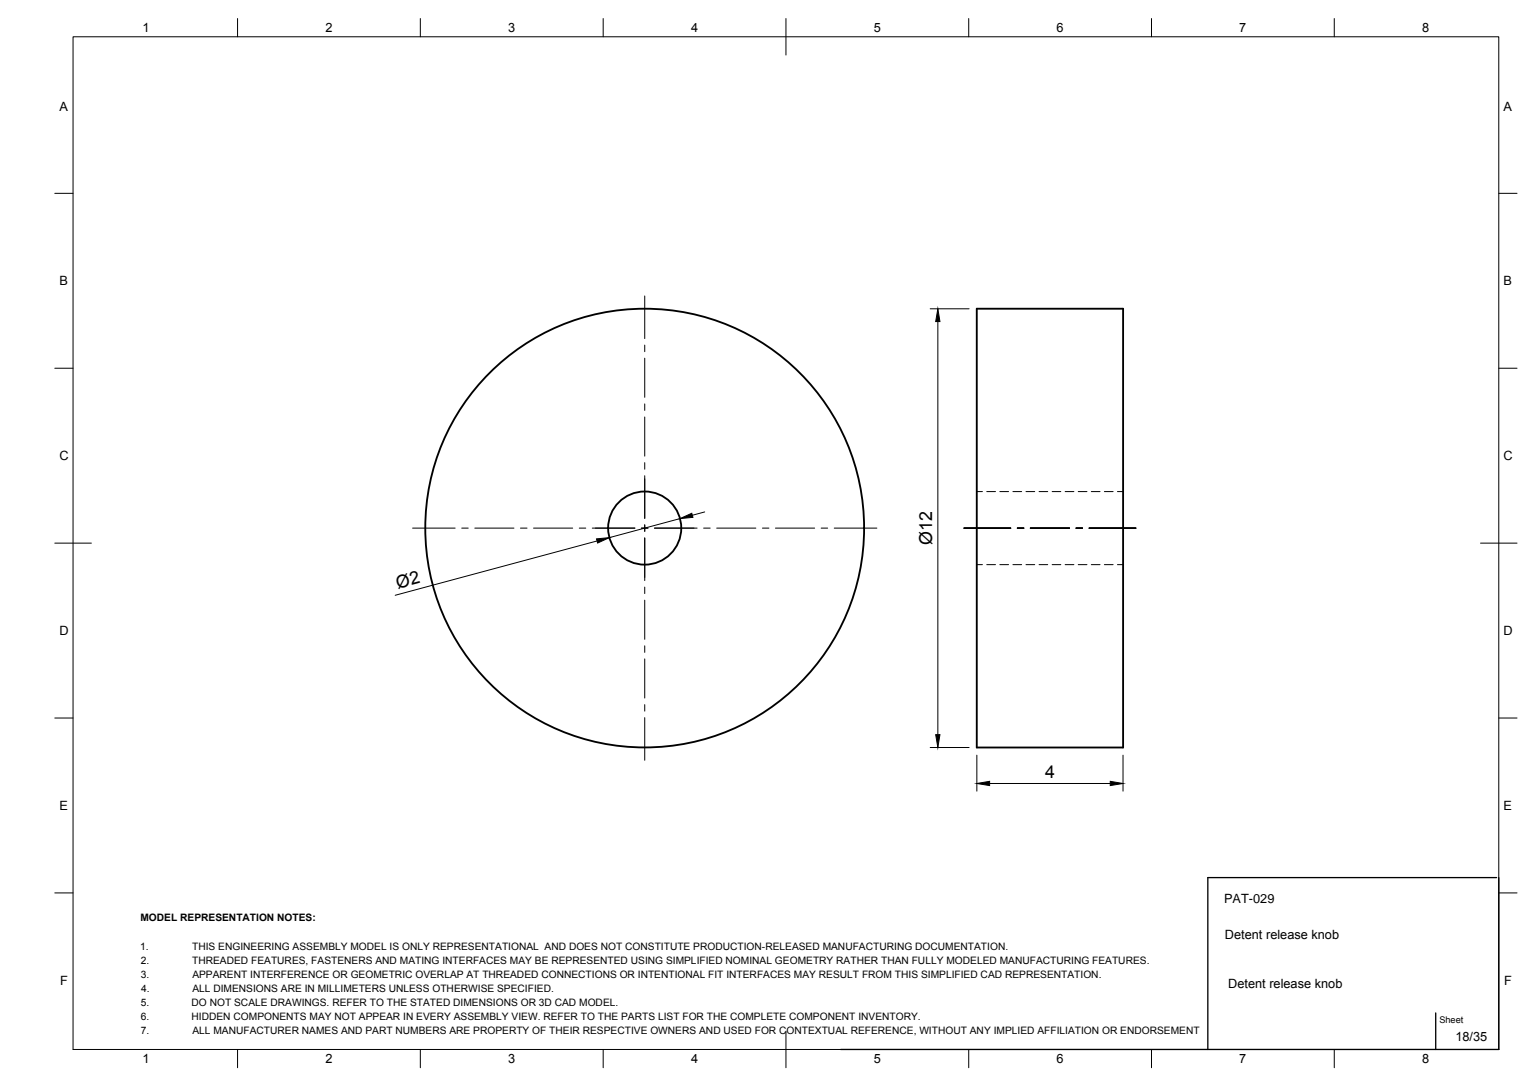
ISO-10303-21;
HEADER;
/* Generated by software containing ST-Developer
 * from STEP Tools, Inc. (www.steptools.com) 
 */

FILE_DESCRIPTION(
/* description */ ('Door-style hinge test fixture with detent'),
/* implementation_level */ '2;1');

FILE_NAME(
/* name */ 'Detent release knob.step',
/* time_stamp */ '2026-10-28T03:24:57-07:00',
/* author */ (''),
/* organization */ (''),
/* preprocessor_version */ 'ST-DEVELOPER v20.2',
/* originating_system */ 'Autodesk Translation Framework v15.17.0.0',
/* authorisation */ '');

FILE_SCHEMA (('AUTOMOTIVE_DESIGN { 1 0 10303 214 3 1 1 }'));
ENDSEC;

DATA;
#10=MECHANICAL_DESIGN_GEOMETRIC_PRESENTATION_REPRESENTATION('',(#336),#9813);
#273=SHAPE_REPRESENTATION_RELATIONSHIP('SRR','None',#9950,#304);
#304=ADVANCED_BREP_SHAPE_REPRESENTATION('',(#376),#9793);
#336=STYLED_ITEM('',(#10169),#376);
#376=MANIFOLD_SOLID_BREP('Body1',#4767);
#463=FACE_BOUND('',#1138,.T.);
#464=FACE_BOUND('',#1140,.T.);
#576=PLANE('',#5388);
#577=PLANE('',#5389);
#786=FACE_OUTER_BOUND('',#1135,.T.);
#787=FACE_OUTER_BOUND('',#1136,.T.);
#788=FACE_OUTER_BOUND('',#1137,.T.);
#789=FACE_OUTER_BOUND('',#1139,.T.);
#1135=EDGE_LOOP('',(#3761,#3762,#3763,#3764));
#1136=EDGE_LOOP('',(#3765,#3766,#3767,#3768));
#1137=EDGE_LOOP('',(#3769));
#1138=EDGE_LOOP('',(#3770));
#1139=EDGE_LOOP('',(#3771));
#1140=EDGE_LOOP('',(#3772));
#1506=LINE('',#7903,#1826);
#1507=LINE('',#7909,#1827);
#1826=VECTOR('',#6415,0.1);
#1827=VECTOR('',#6422,0.6);
#2079=CIRCLE('',#5383,0.1);
#2080=CIRCLE('',#5384,0.1);
#2081=CIRCLE('',#5386,0.6);
#2082=CIRCLE('',#5387,0.6);
#2407=VERTEX_POINT('',#7900);
#2408=VERTEX_POINT('',#7902);
#2409=VERTEX_POINT('',#7906);
#2410=VERTEX_POINT('',#7908);
#2897=EDGE_CURVE('',#2407,#2407,#2079,.T.);
#2898=EDGE_CURVE('',#2407,#2408,#1506,.T.);
#2899=EDGE_CURVE('',#2408,#2408,#2080,.T.);
#2900=EDGE_CURVE('',#2409,#2409,#2081,.T.);
#2901=EDGE_CURVE('',#2409,#2410,#1507,.T.);
#2902=EDGE_CURVE('',#2410,#2410,#2082,.T.);
#3761=ORIENTED_EDGE('',*,*,#2897,.F.);
#3762=ORIENTED_EDGE('',*,*,#2898,.T.);
#3763=ORIENTED_EDGE('',*,*,#2899,.T.);
#3764=ORIENTED_EDGE('',*,*,#2898,.F.);
#3765=ORIENTED_EDGE('',*,*,#2900,.F.);
#3766=ORIENTED_EDGE('',*,*,#2901,.T.);
#3767=ORIENTED_EDGE('',*,*,#2902,.T.);
#3768=ORIENTED_EDGE('',*,*,#2901,.F.);
#3769=ORIENTED_EDGE('',*,*,#2900,.T.);
#3770=ORIENTED_EDGE('',*,*,#2897,.T.);
#3771=ORIENTED_EDGE('',*,*,#2902,.F.);
#3772=ORIENTED_EDGE('',*,*,#2899,.F.);
#4427=CYLINDRICAL_SURFACE('',#5382,0.1);
#4428=CYLINDRICAL_SURFACE('',#5385,0.6);
#4591=ADVANCED_FACE('',(#786),#4427,.F.);
#4592=ADVANCED_FACE('',(#787),#4428,.T.);
#4593=ADVANCED_FACE('',(#788,#463),#576,.T.);
#4594=ADVANCED_FACE('',(#789,#464),#577,.F.);
#4767=CLOSED_SHELL('',(#4591,#4592,#4593,#4594));
#5381=AXIS2_PLACEMENT_3D('',#7898,#6409,#6410);
#5382=AXIS2_PLACEMENT_3D('',#7899,#6411,#6412);
#5383=AXIS2_PLACEMENT_3D('',#7901,#6413,#6414);
#5384=AXIS2_PLACEMENT_3D('',#7904,#6416,#6417);
#5385=AXIS2_PLACEMENT_3D('',#7905,#6418,#6419);
#5386=AXIS2_PLACEMENT_3D('',#7907,#6420,#6421);
#5387=AXIS2_PLACEMENT_3D('',#7910,#6423,#6424);
#5388=AXIS2_PLACEMENT_3D('',#7911,#6425,#6426);
#5389=AXIS2_PLACEMENT_3D('',#7912,#6427,#6428);
#6409=DIRECTION('axis',(0.,0.,1.));
#6410=DIRECTION('refdir',(1.,0.,0.));
#6411=DIRECTION('center_axis',(0.,1.,0.));
#6412=DIRECTION('ref_axis',(1.,0.,0.));
#6413=DIRECTION('center_axis',(0.,-1.,0.));
#6414=DIRECTION('ref_axis',(1.,0.,0.));
#6415=DIRECTION('',(0.,-1.,0.));
#6416=DIRECTION('center_axis',(0.,-1.,0.));
#6417=DIRECTION('ref_axis',(1.,0.,0.));
#6418=DIRECTION('center_axis',(0.,1.,0.));
#6419=DIRECTION('ref_axis',(1.,0.,0.));
#6420=DIRECTION('center_axis',(0.,1.,0.));
#6421=DIRECTION('ref_axis',(1.,0.,0.));
#6422=DIRECTION('',(0.,-1.,0.));
#6423=DIRECTION('center_axis',(0.,1.,0.));
#6424=DIRECTION('ref_axis',(1.,0.,0.));
#6425=DIRECTION('center_axis',(0.,1.,0.));
#6426=DIRECTION('ref_axis',(1.,0.,0.));
#6427=DIRECTION('center_axis',(0.,1.,0.));
#6428=DIRECTION('ref_axis',(1.,0.,0.));
#7898=CARTESIAN_POINT('',(0.,0.,0.));
#7899=CARTESIAN_POINT('Origin',(0.,-5.,7.2));
#7900=CARTESIAN_POINT('',(-0.1,-4.6,7.2));
#7901=CARTESIAN_POINT('Origin',(0.,-4.6,7.2));
#7902=CARTESIAN_POINT('',(-0.1,-5.,7.2));
#7903=CARTESIAN_POINT('',(-0.1,-5.,7.2));
#7904=CARTESIAN_POINT('Origin',(0.,-5.,7.2));
#7905=CARTESIAN_POINT('Origin',(0.,-5.,7.2));
#7906=CARTESIAN_POINT('',(-0.6,-4.6,7.2));
#7907=CARTESIAN_POINT('Origin',(0.,-4.6,7.2));
#7908=CARTESIAN_POINT('',(-0.6,-5.,7.2));
#7909=CARTESIAN_POINT('',(-0.6,-5.,7.2));
#7910=CARTESIAN_POINT('Origin',(0.,-5.,7.2));
#7911=CARTESIAN_POINT('Origin',(0.,-4.6,7.2));
#7912=CARTESIAN_POINT('Origin',(0.,-5.,7.2));
#9757=UNCERTAINTY_MEASURE_WITH_UNIT(LENGTH_MEASURE(0.001),#9814,
'DISTANCE_ACCURACY_VALUE',
'Maximum model space distance between geometric entities at asserted c
onnectivities');
#9777=UNCERTAINTY_MEASURE_WITH_UNIT(LENGTH_MEASURE(0.001),#9814,
'DISTANCE_ACCURACY_VALUE',
'Maximum model space distance between geometric entities at asserted c
onnectivities');
#9793=(
GEOMETRIC_REPRESENTATION_CONTEXT(3)
GLOBAL_UNCERTAINTY_ASSIGNED_CONTEXT((#9757))
GLOBAL_UNIT_ASSIGNED_CONTEXT((#9814,#9816,#9817))
REPRESENTATION_CONTEXT('','3D')
);
#9813=(
GEOMETRIC_REPRESENTATION_CONTEXT(3)
GLOBAL_UNCERTAINTY_ASSIGNED_CONTEXT((#9777))
GLOBAL_UNIT_ASSIGNED_CONTEXT((#9814,#9816,#9817))
REPRESENTATION_CONTEXT('','3D')
);
#9814=(
LENGTH_UNIT()
NAMED_UNIT(*)
SI_UNIT(.CENTI.,.METRE.)
);
#9816=(
NAMED_UNIT(*)
PLANE_ANGLE_UNIT()
SI_UNIT($,.RADIAN.)
);
#9817=(
NAMED_UNIT(*)
SI_UNIT($,.STERADIAN.)
SOLID_ANGLE_UNIT()
);
#9833=SHAPE_DEFINITION_REPRESENTATION(#9868,#9950);
#9868=PRODUCT_DEFINITION_SHAPE('',$,#9986);
#9950=SHAPE_REPRESENTATION('',(#5381),#9793);
#9970=PRODUCT_DEFINITION_CONTEXT('part definition',#10077,'design');
#9986=PRODUCT_DEFINITION('Detent release knob','Detent release knob',#10021,
#9970);
#10021=PRODUCT_DEFINITION_FORMATION('',$,#10094);
#10077=APPLICATION_CONTEXT(
'Core Data for Automotive Mechanical Design Process');
#10078=PRODUCT_CONTEXT('part definition',#10077,'mechanical');
#10094=PRODUCT('Detent release knob','Detent release knob',
'Detent release knob',(#10078));
#10163=COLOUR_RGB('Light Blue',0.38,0.62,0.78);
#10164=FILL_AREA_STYLE_COLOUR('',#10163);
#10165=FILL_AREA_STYLE('',(#10164));
#10166=SURFACE_STYLE_FILL_AREA(#10165);
#10167=SURFACE_SIDE_STYLE('',(#10166));
#10168=SURFACE_STYLE_USAGE(.BOTH.,#10167);
#10169=PRESENTATION_STYLE_ASSIGNMENT((#10168));
ENDSEC;
END-ISO-10303-21;
